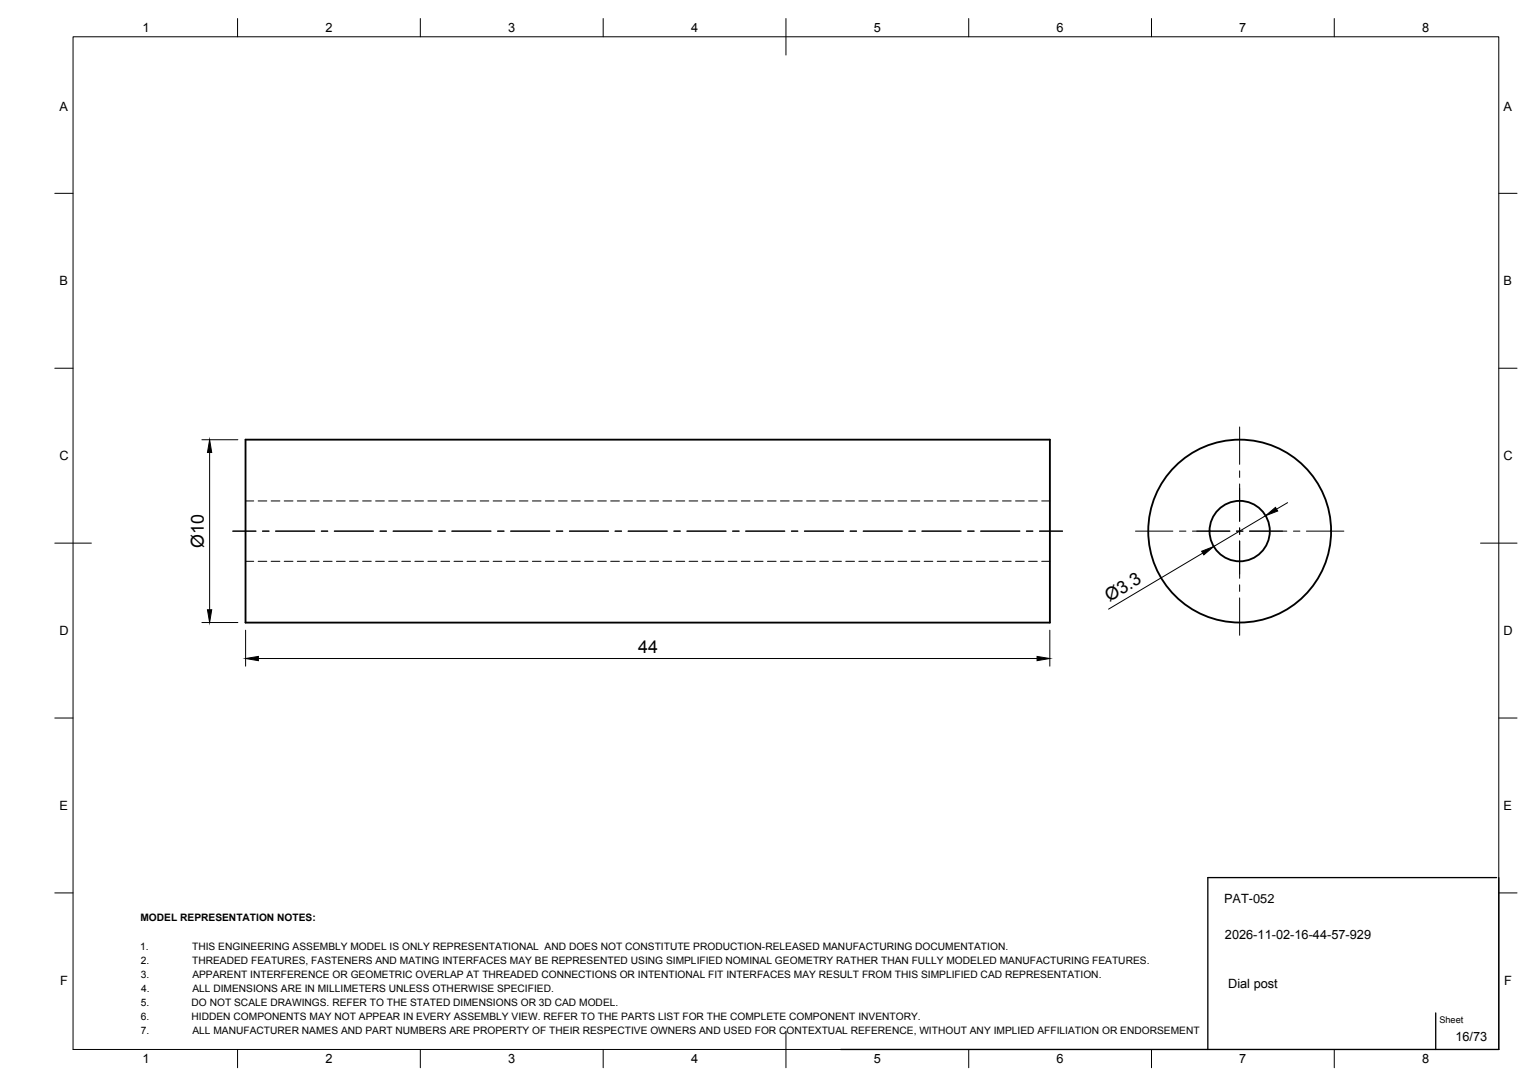
ISO-10303-21;
HEADER;
/* Generated by software containing ST-Developer
 * from STEP Tools, Inc. (www.steptools.com) 
 */

FILE_DESCRIPTION(
/* description */ ('Hand-crank gear train demonstrator'),
/* implementation_level */ '2;1');

FILE_NAME(
/* name */ 'Dial post.step',
/* time_stamp */ '2026-10-28T03:22:13-07:00',
/* author */ (''),
/* organization */ (''),
/* preprocessor_version */ 'ST-DEVELOPER v20.2',
/* originating_system */ 'Autodesk Translation Framework v15.17.0.0',
/* authorisation */ '');

FILE_SCHEMA (('AUTOMOTIVE_DESIGN { 1 0 10303 214 3 1 1 }'));
ENDSEC;

DATA;
#10=MECHANICAL_DESIGN_GEOMETRIC_PRESENTATION_REPRESENTATION('',(#1227),#62758);
#1084=SHAPE_REPRESENTATION_RELATIONSHIP('SRR','None',#63058,#1148);
#1148=ADVANCED_BREP_SHAPE_REPRESENTATION('',(#1304),#62712);
#1227=STYLED_ITEM('',(#63455),#1304);
#1304=MANIFOLD_SOLID_BREP('Body1',#16409);
#1536=FACE_BOUND('',#3642,.T.);
#1537=FACE_BOUND('',#3644,.T.);
#1855=PLANE('',#17919);
#1856=PLANE('',#17920);
#2509=FACE_OUTER_BOUND('',#3639,.T.);
#2510=FACE_OUTER_BOUND('',#3640,.T.);
#2511=FACE_OUTER_BOUND('',#3641,.T.);
#2512=FACE_OUTER_BOUND('',#3643,.T.);
#3639=EDGE_LOOP('',(#12571,#12572,#12573,#12574));
#3640=EDGE_LOOP('',(#12575,#12576,#12577,#12578));
#3641=EDGE_LOOP('',(#12579));
#3642=EDGE_LOOP('',(#12580));
#3643=EDGE_LOOP('',(#12581));
#3644=EDGE_LOOP('',(#12582));
#4791=LINE('',#25831,#5923);
#4792=LINE('',#25837,#5924);
#5923=VECTOR('',#20850,0.164999999999999);
#5924=VECTOR('',#20857,0.5);
#6881=CIRCLE('',#17914,0.164999999999999);
#6882=CIRCLE('',#17915,0.164999999999999);
#6883=CIRCLE('',#17917,0.5);
#6884=CIRCLE('',#17918,0.5);
#7806=VERTEX_POINT('',#25828);
#7807=VERTEX_POINT('',#25830);
#7808=VERTEX_POINT('',#25834);
#7809=VERTEX_POINT('',#25836);
#9537=EDGE_CURVE('',#7806,#7806,#6881,.T.);
#9538=EDGE_CURVE('',#7806,#7807,#4791,.T.);
#9539=EDGE_CURVE('',#7807,#7807,#6882,.T.);
#9540=EDGE_CURVE('',#7808,#7808,#6883,.T.);
#9541=EDGE_CURVE('',#7808,#7809,#4792,.T.);
#9542=EDGE_CURVE('',#7809,#7809,#6884,.T.);
#12571=ORIENTED_EDGE('',*,*,#9537,.F.);
#12572=ORIENTED_EDGE('',*,*,#9538,.T.);
#12573=ORIENTED_EDGE('',*,*,#9539,.F.);
#12574=ORIENTED_EDGE('',*,*,#9538,.F.);
#12575=ORIENTED_EDGE('',*,*,#9540,.F.);
#12576=ORIENTED_EDGE('',*,*,#9541,.T.);
#12577=ORIENTED_EDGE('',*,*,#9542,.T.);
#12578=ORIENTED_EDGE('',*,*,#9541,.F.);
#12579=ORIENTED_EDGE('',*,*,#9540,.T.);
#12580=ORIENTED_EDGE('',*,*,#9539,.T.);
#12581=ORIENTED_EDGE('',*,*,#9542,.F.);
#12582=ORIENTED_EDGE('',*,*,#9537,.T.);
#15283=CYLINDRICAL_SURFACE('',#17913,0.164999999999999);
#15284=CYLINDRICAL_SURFACE('',#17916,0.5);
#15819=ADVANCED_FACE('',(#2509),#15283,.F.);
#15820=ADVANCED_FACE('',(#2510),#15284,.T.);
#15821=ADVANCED_FACE('',(#2511,#1536),#1855,.T.);
#15822=ADVANCED_FACE('',(#2512,#1537),#1856,.F.);
#16409=CLOSED_SHELL('',(#15819,#15820,#15821,#15822));
#17912=AXIS2_PLACEMENT_3D('',#25826,#20844,#20845);
#17913=AXIS2_PLACEMENT_3D('',#25827,#20846,#20847);
#17914=AXIS2_PLACEMENT_3D('',#25829,#20848,#20849);
#17915=AXIS2_PLACEMENT_3D('',#25832,#20851,#20852);
#17916=AXIS2_PLACEMENT_3D('',#25833,#20853,#20854);
#17917=AXIS2_PLACEMENT_3D('',#25835,#20855,#20856);
#17918=AXIS2_PLACEMENT_3D('',#25838,#20858,#20859);
#17919=AXIS2_PLACEMENT_3D('',#25839,#20860,#20861);
#17920=AXIS2_PLACEMENT_3D('',#25840,#20862,#20863);
#20844=DIRECTION('axis',(0.,0.,1.));
#20845=DIRECTION('refdir',(1.,0.,0.));
#20846=DIRECTION('center_axis',(0.,1.,0.));
#20847=DIRECTION('ref_axis',(1.,0.,0.));
#20848=DIRECTION('center_axis',(0.,1.,0.));
#20849=DIRECTION('ref_axis',(1.,0.,0.));
#20850=DIRECTION('',(0.,1.,0.));
#20851=DIRECTION('center_axis',(0.,-1.,0.));
#20852=DIRECTION('ref_axis',(1.,0.,0.));
#20853=DIRECTION('center_axis',(0.,1.,0.));
#20854=DIRECTION('ref_axis',(1.,0.,0.));
#20855=DIRECTION('center_axis',(0.,1.,0.));
#20856=DIRECTION('ref_axis',(1.,0.,0.));
#20857=DIRECTION('',(0.,-1.,0.));
#20858=DIRECTION('center_axis',(0.,1.,0.));
#20859=DIRECTION('ref_axis',(1.,0.,0.));
#20860=DIRECTION('center_axis',(0.,1.,0.));
#20861=DIRECTION('ref_axis',(1.,0.,0.));
#20862=DIRECTION('center_axis',(0.,1.,0.));
#20863=DIRECTION('ref_axis',(1.,0.,0.));
#25826=CARTESIAN_POINT('',(0.,0.,0.));
#25827=CARTESIAN_POINT('Origin',(23.,-0.7,4.));
#25828=CARTESIAN_POINT('',(22.835,-0.6,4.));
#25829=CARTESIAN_POINT('Origin',(23.,-0.6,4.));
#25830=CARTESIAN_POINT('',(22.835,3.8,4.));
#25831=CARTESIAN_POINT('',(22.835,-0.7,4.));
#25832=CARTESIAN_POINT('Origin',(23.,3.8,4.));
#25833=CARTESIAN_POINT('Origin',(23.,-0.6,4.));
#25834=CARTESIAN_POINT('',(22.5,3.8,4.));
#25835=CARTESIAN_POINT('Origin',(23.,3.8,4.));
#25836=CARTESIAN_POINT('',(22.5,-0.6,4.));
#25837=CARTESIAN_POINT('',(22.5,-0.6,4.));
#25838=CARTESIAN_POINT('Origin',(23.,-0.6,4.));
#25839=CARTESIAN_POINT('Origin',(23.,3.8,4.));
#25840=CARTESIAN_POINT('Origin',(23.,-0.6,4.));
#62638=UNCERTAINTY_MEASURE_WITH_UNIT(LENGTH_MEASURE(0.001),#62759,
'DISTANCE_ACCURACY_VALUE',
'Maximum model space distance between geometric entities at asserted c
onnectivities');
#62684=UNCERTAINTY_MEASURE_WITH_UNIT(LENGTH_MEASURE(0.001),#62759,
'DISTANCE_ACCURACY_VALUE',
'Maximum model space distance between geometric entities at asserted c
onnectivities');
#62712=(
GEOMETRIC_REPRESENTATION_CONTEXT(3)
GLOBAL_UNCERTAINTY_ASSIGNED_CONTEXT((#62638))
GLOBAL_UNIT_ASSIGNED_CONTEXT((#62759,#62761,#62762))
REPRESENTATION_CONTEXT('','3D')
);
#62758=(
GEOMETRIC_REPRESENTATION_CONTEXT(3)
GLOBAL_UNCERTAINTY_ASSIGNED_CONTEXT((#62684))
GLOBAL_UNIT_ASSIGNED_CONTEXT((#62759,#62761,#62762))
REPRESENTATION_CONTEXT('','3D')
);
#62759=(
LENGTH_UNIT()
NAMED_UNIT(*)
SI_UNIT(.CENTI.,.METRE.)
);
#62761=(
NAMED_UNIT(*)
PLANE_ANGLE_UNIT()
SI_UNIT($,.RADIAN.)
);
#62762=(
NAMED_UNIT(*)
SI_UNIT($,.STERADIAN.)
SOLID_ANGLE_UNIT()
);
#62790=SHAPE_DEFINITION_REPRESENTATION(#62873,#63058);
#62873=PRODUCT_DEFINITION_SHAPE('',$,#63132);
#63058=SHAPE_REPRESENTATION('',(#17912),#62712);
#63104=PRODUCT_DEFINITION_CONTEXT('part definition',#63325,'design');
#63132=PRODUCT_DEFINITION('Dial post','Dial post',#63205,#63104);
#63205=PRODUCT_DEFINITION_FORMATION('',$,#63354);
#63325=APPLICATION_CONTEXT(
'Core Data for Automotive Mechanical Design Process');
#63326=PRODUCT_CONTEXT('part definition',#63325,'mechanical');
#63354=PRODUCT('Dial post','Dial post','Dial post',(#63326));
#63449=COLOUR_RGB('Sky Blue',0.24,0.69,0.87);
#63450=FILL_AREA_STYLE_COLOUR('',#63449);
#63451=FILL_AREA_STYLE('',(#63450));
#63452=SURFACE_STYLE_FILL_AREA(#63451);
#63453=SURFACE_SIDE_STYLE('',(#63452));
#63454=SURFACE_STYLE_USAGE(.BOTH.,#63453);
#63455=PRESENTATION_STYLE_ASSIGNMENT((#63454));
ENDSEC;
END-ISO-10303-21;
